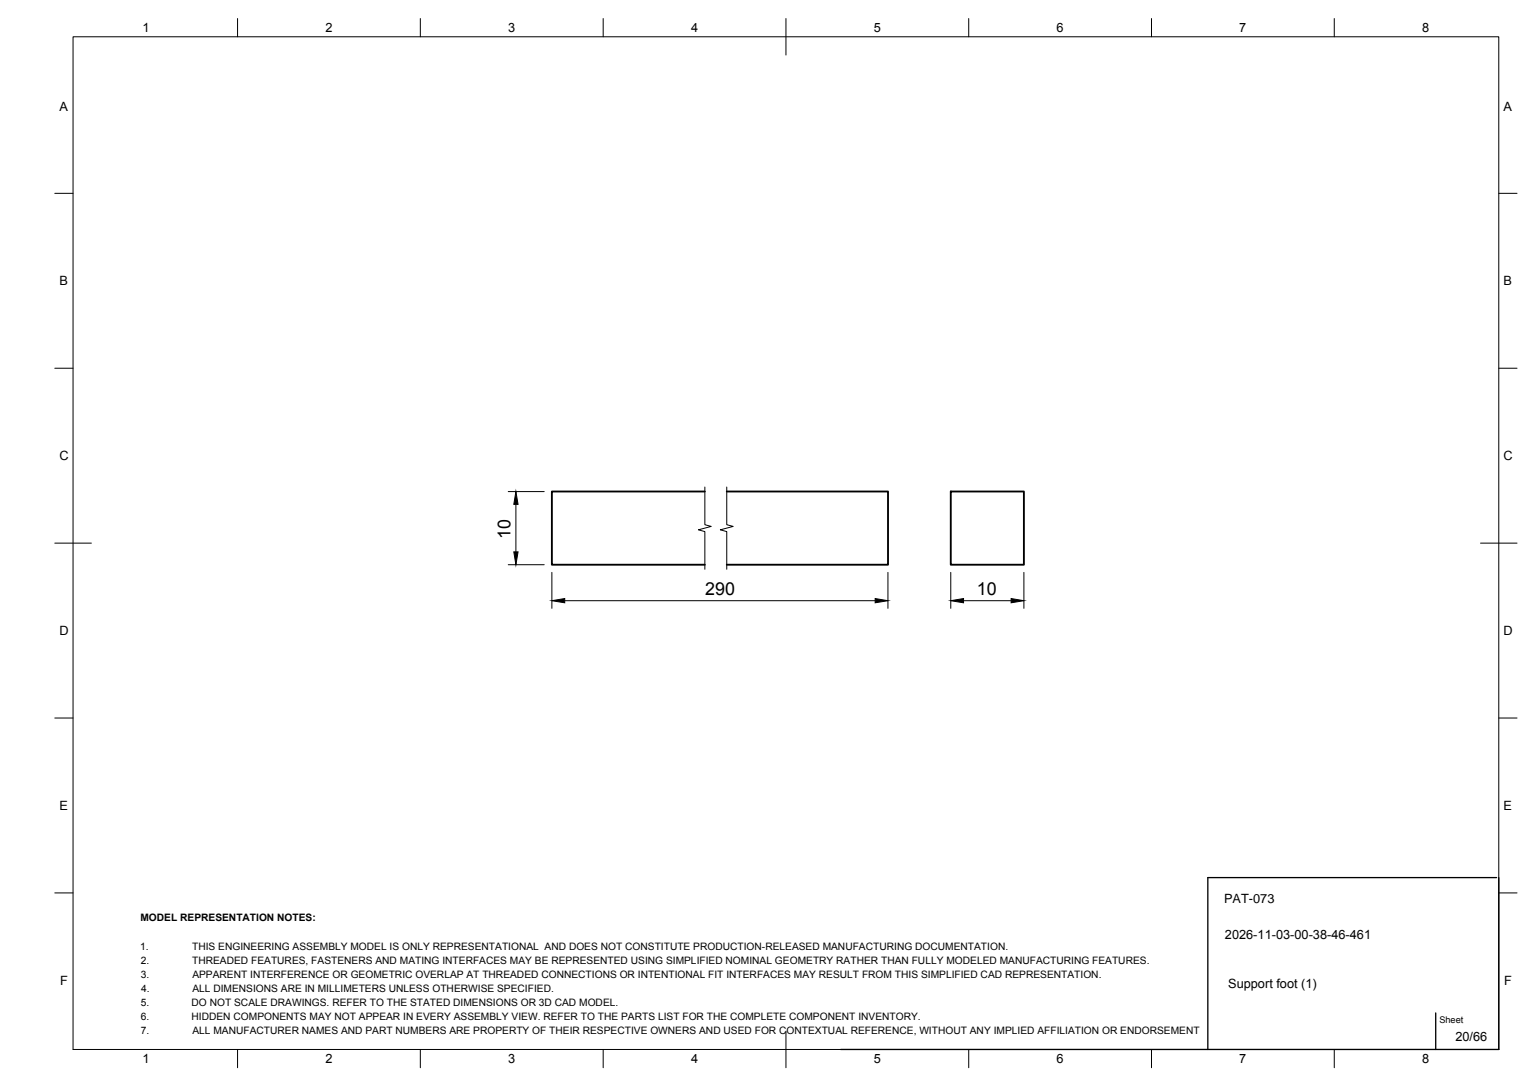
ISO-10303-21;
HEADER;
/* Generated by software containing ST-Developer
 * from STEP Tools, Inc. (www.steptools.com) 
 */

FILE_DESCRIPTION(
/* description */ ('Manual piston pump'),
/* implementation_level */ '2;1');

FILE_NAME(
/* name */ 'Support foot (1).step',
/* time_stamp */ '2026-11-02T16:54:23-08:00',
/* author */ (''),
/* organization */ (''),
/* preprocessor_version */ 'ST-DEVELOPER v20.2',
/* originating_system */ 'Autodesk Translation Framework v15.17.0.0',
/* authorisation */ '');

FILE_SCHEMA (('AUTOMOTIVE_DESIGN { 1 0 10303 214 3 1 1 }'));
ENDSEC;

DATA;
#10=MECHANICAL_DESIGN_GEOMETRIC_PRESENTATION_REPRESENTATION('',(#706),#19043);
#580=SHAPE_REPRESENTATION_RELATIONSHIP('SRR','None',#19326,#643);
#643=ADVANCED_BREP_SHAPE_REPRESENTATION('',(#777),#18993);
#706=STYLED_ITEM('',(#19662),#777);
#777=MANIFOLD_SOLID_BREP('Body1',#9491);
#1462=FACE_OUTER_BOUND('',#2111,.T.);
#1463=FACE_OUTER_BOUND('',#2112,.T.);
#1464=FACE_OUTER_BOUND('',#2113,.T.);
#1465=FACE_OUTER_BOUND('',#2114,.T.);
#1466=FACE_OUTER_BOUND('',#2115,.T.);
#1467=FACE_OUTER_BOUND('',#2116,.T.);
#2111=EDGE_LOOP('',(#6961,#6962,#6963,#6964));
#2112=EDGE_LOOP('',(#6965,#6966,#6967,#6968));
#2113=EDGE_LOOP('',(#6969,#6970,#6971,#6972));
#2114=EDGE_LOOP('',(#6973,#6974,#6975,#6976));
#2115=EDGE_LOOP('',(#6977,#6978,#6979,#6980));
#2116=EDGE_LOOP('',(#6981,#6982,#6983,#6984));
#3337=LINE('',#15442,#3941);
#3338=LINE('',#15444,#3942);
#3339=LINE('',#15446,#3943);
#3340=LINE('',#15447,#3944);
#3341=LINE('',#15450,#3945);
#3342=LINE('',#15452,#3946);
#3343=LINE('',#15453,#3947);
#3344=LINE('',#15456,#3948);
#3345=LINE('',#15458,#3949);
#3346=LINE('',#15459,#3950);
#3347=LINE('',#15461,#3951);
#3348=LINE('',#15462,#3952);
#3941=VECTOR('',#12347,1.);
#3942=VECTOR('',#12348,1.);
#3943=VECTOR('',#12349,1.);
#3944=VECTOR('',#12350,1.);
#3945=VECTOR('',#12353,1.);
#3946=VECTOR('',#12354,1.);
#3947=VECTOR('',#12355,1.);
#3948=VECTOR('',#12358,1.);
#3949=VECTOR('',#12359,1.);
#3950=VECTOR('',#12360,1.);
#3951=VECTOR('',#12363,1.);
#3952=VECTOR('',#12364,1.);
#4581=VERTEX_POINT('',#15440);
#4582=VERTEX_POINT('',#15441);
#4583=VERTEX_POINT('',#15443);
#4584=VERTEX_POINT('',#15445);
#4585=VERTEX_POINT('',#15449);
#4586=VERTEX_POINT('',#15451);
#4587=VERTEX_POINT('',#15455);
#4588=VERTEX_POINT('',#15457);
#5467=EDGE_CURVE('',#4581,#4582,#3337,.T.);
#5468=EDGE_CURVE('',#4582,#4583,#3338,.T.);
#5469=EDGE_CURVE('',#4584,#4583,#3339,.T.);
#5470=EDGE_CURVE('',#4581,#4584,#3340,.T.);
#5471=EDGE_CURVE('',#4585,#4581,#3341,.T.);
#5472=EDGE_CURVE('',#4586,#4584,#3342,.T.);
#5473=EDGE_CURVE('',#4585,#4586,#3343,.T.);
#5474=EDGE_CURVE('',#4587,#4585,#3344,.T.);
#5475=EDGE_CURVE('',#4588,#4586,#3345,.T.);
#5476=EDGE_CURVE('',#4587,#4588,#3346,.T.);
#5477=EDGE_CURVE('',#4582,#4587,#3347,.T.);
#5478=EDGE_CURVE('',#4583,#4588,#3348,.T.);
#6961=ORIENTED_EDGE('',*,*,#5467,.T.);
#6962=ORIENTED_EDGE('',*,*,#5468,.T.);
#6963=ORIENTED_EDGE('',*,*,#5469,.F.);
#6964=ORIENTED_EDGE('',*,*,#5470,.F.);
#6965=ORIENTED_EDGE('',*,*,#5471,.T.);
#6966=ORIENTED_EDGE('',*,*,#5470,.T.);
#6967=ORIENTED_EDGE('',*,*,#5472,.F.);
#6968=ORIENTED_EDGE('',*,*,#5473,.F.);
#6969=ORIENTED_EDGE('',*,*,#5474,.T.);
#6970=ORIENTED_EDGE('',*,*,#5473,.T.);
#6971=ORIENTED_EDGE('',*,*,#5475,.F.);
#6972=ORIENTED_EDGE('',*,*,#5476,.F.);
#6973=ORIENTED_EDGE('',*,*,#5477,.T.);
#6974=ORIENTED_EDGE('',*,*,#5476,.T.);
#6975=ORIENTED_EDGE('',*,*,#5478,.F.);
#6976=ORIENTED_EDGE('',*,*,#5468,.F.);
#6977=ORIENTED_EDGE('',*,*,#5478,.T.);
#6978=ORIENTED_EDGE('',*,*,#5475,.T.);
#6979=ORIENTED_EDGE('',*,*,#5472,.T.);
#6980=ORIENTED_EDGE('',*,*,#5469,.T.);
#6981=ORIENTED_EDGE('',*,*,#5477,.F.);
#6982=ORIENTED_EDGE('',*,*,#5467,.F.);
#6983=ORIENTED_EDGE('',*,*,#5471,.F.);
#6984=ORIENTED_EDGE('',*,*,#5474,.F.);
#8671=PLANE('',#10573);
#8672=PLANE('',#10574);
#8673=PLANE('',#10575);
#8674=PLANE('',#10576);
#8675=PLANE('',#10577);
#8676=PLANE('',#10578);
#9067=ADVANCED_FACE('',(#1462),#8671,.T.);
#9068=ADVANCED_FACE('',(#1463),#8672,.T.);
#9069=ADVANCED_FACE('',(#1464),#8673,.T.);
#9070=ADVANCED_FACE('',(#1465),#8674,.T.);
#9071=ADVANCED_FACE('',(#1466),#8675,.T.);
#9072=ADVANCED_FACE('',(#1467),#8676,.F.);
#9491=CLOSED_SHELL('',(#9067,#9068,#9069,#9070,#9071,#9072));
#10572=AXIS2_PLACEMENT_3D('',#15438,#12343,#12344);
#10573=AXIS2_PLACEMENT_3D('',#15439,#12345,#12346);
#10574=AXIS2_PLACEMENT_3D('',#15448,#12351,#12352);
#10575=AXIS2_PLACEMENT_3D('',#15454,#12356,#12357);
#10576=AXIS2_PLACEMENT_3D('',#15460,#12361,#12362);
#10577=AXIS2_PLACEMENT_3D('',#15463,#12365,#12366);
#10578=AXIS2_PLACEMENT_3D('',#15464,#12367,#12368);
#12343=DIRECTION('axis',(0.,0.,1.));
#12344=DIRECTION('refdir',(1.,0.,0.));
#12345=DIRECTION('center_axis',(0.,1.,0.));
#12346=DIRECTION('ref_axis',(-1.,0.,0.));
#12347=DIRECTION('',(-1.,0.,0.));
#12348=DIRECTION('',(0.,0.,1.));
#12349=DIRECTION('',(-1.,0.,0.));
#12350=DIRECTION('',(0.,0.,1.));
#12351=DIRECTION('center_axis',(1.,0.,0.));
#12352=DIRECTION('ref_axis',(0.,1.,0.));
#12353=DIRECTION('',(0.,1.,0.));
#12354=DIRECTION('',(0.,1.,0.));
#12355=DIRECTION('',(0.,0.,1.));
#12356=DIRECTION('center_axis',(0.,-1.,0.));
#12357=DIRECTION('ref_axis',(1.,0.,0.));
#12358=DIRECTION('',(1.,0.,0.));
#12359=DIRECTION('',(1.,0.,0.));
#12360=DIRECTION('',(0.,0.,1.));
#12361=DIRECTION('center_axis',(-1.,0.,0.));
#12362=DIRECTION('ref_axis',(0.,-1.,0.));
#12363=DIRECTION('',(0.,-1.,0.));
#12364=DIRECTION('',(0.,-1.,0.));
#12365=DIRECTION('center_axis',(0.,0.,1.));
#12366=DIRECTION('ref_axis',(1.,0.,0.));
#12367=DIRECTION('center_axis',(0.,0.,1.));
#12368=DIRECTION('ref_axis',(1.,0.,0.));
#15438=CARTESIAN_POINT('',(0.,0.,0.));
#15439=CARTESIAN_POINT('Origin',(8.5,15.,-2.));
#15440=CARTESIAN_POINT('',(8.5,15.,-2.));
#15441=CARTESIAN_POINT('',(7.5,15.,-2.));
#15442=CARTESIAN_POINT('',(8.5,15.,-2.));
#15443=CARTESIAN_POINT('',(7.5,15.,-1.));
#15444=CARTESIAN_POINT('',(7.5,15.,-2.));
#15445=CARTESIAN_POINT('',(8.5,15.,-1.));
#15446=CARTESIAN_POINT('',(8.5,15.,-1.));
#15447=CARTESIAN_POINT('',(8.5,15.,-2.));
#15448=CARTESIAN_POINT('Origin',(8.5,-14.,-2.));
#15449=CARTESIAN_POINT('',(8.5,-14.,-2.));
#15450=CARTESIAN_POINT('',(8.5,-14.,-2.));
#15451=CARTESIAN_POINT('',(8.5,-14.,-1.));
#15452=CARTESIAN_POINT('',(8.5,-14.,-1.));
#15453=CARTESIAN_POINT('',(8.5,-14.,-2.));
#15454=CARTESIAN_POINT('Origin',(7.5,-14.,-2.));
#15455=CARTESIAN_POINT('',(7.5,-14.,-2.));
#15456=CARTESIAN_POINT('',(7.5,-14.,-2.));
#15457=CARTESIAN_POINT('',(7.5,-14.,-1.));
#15458=CARTESIAN_POINT('',(7.5,-14.,-1.));
#15459=CARTESIAN_POINT('',(7.5,-14.,-2.));
#15460=CARTESIAN_POINT('Origin',(7.5,15.,-2.));
#15461=CARTESIAN_POINT('',(7.5,15.,-2.));
#15462=CARTESIAN_POINT('',(7.5,15.,-1.));
#15463=CARTESIAN_POINT('Origin',(8.,0.5,-1.));
#15464=CARTESIAN_POINT('Origin',(8.,0.5,-2.));
#18922=UNCERTAINTY_MEASURE_WITH_UNIT(LENGTH_MEASURE(0.001),#19044,
'DISTANCE_ACCURACY_VALUE',
'Maximum model space distance between geometric entities at asserted c
onnectivities');
#18972=UNCERTAINTY_MEASURE_WITH_UNIT(LENGTH_MEASURE(0.001),#19044,
'DISTANCE_ACCURACY_VALUE',
'Maximum model space distance between geometric entities at asserted c
onnectivities');
#18993=(
GEOMETRIC_REPRESENTATION_CONTEXT(3)
GLOBAL_UNCERTAINTY_ASSIGNED_CONTEXT((#18922))
GLOBAL_UNIT_ASSIGNED_CONTEXT((#19044,#19046,#19047))
REPRESENTATION_CONTEXT('','3D')
);
#19043=(
GEOMETRIC_REPRESENTATION_CONTEXT(3)
GLOBAL_UNCERTAINTY_ASSIGNED_CONTEXT((#18972))
GLOBAL_UNIT_ASSIGNED_CONTEXT((#19044,#19046,#19047))
REPRESENTATION_CONTEXT('','3D')
);
#19044=(
LENGTH_UNIT()
NAMED_UNIT(*)
SI_UNIT(.CENTI.,.METRE.)
);
#19046=(
NAMED_UNIT(*)
PLANE_ANGLE_UNIT()
SI_UNIT($,.RADIAN.)
);
#19047=(
NAMED_UNIT(*)
SI_UNIT($,.STERADIAN.)
SOLID_ANGLE_UNIT()
);
#19068=SHAPE_DEFINITION_REPRESENTATION(#19138,#19326);
#19138=PRODUCT_DEFINITION_SHAPE('',$,#19397);
#19326=SHAPE_REPRESENTATION('',(#10572),#18993);
#19376=PRODUCT_DEFINITION_CONTEXT('part definition',#19588,'design');
#19397=PRODUCT_DEFINITION('2026-11-03-00-38-46-461','Support foot (1)',
#19467,#19376);
#19467=PRODUCT_DEFINITION_FORMATION('',$,#19610);
#19588=APPLICATION_CONTEXT(
'Core Data for Automotive Mechanical Design Process');
#19589=PRODUCT_CONTEXT('part definition',#19588,'mechanical');
#19610=PRODUCT('2026-11-03-00-38-46-461','Support foot (1)',
'Support foot',(#19589));
#19662=PRESENTATION_STYLE_ASSIGNMENT((#19668));
#19668=SURFACE_STYLE_USAGE(.BOTH.,#19674);
#19674=SURFACE_SIDE_STYLE('',(#19680));
#19680=SURFACE_STYLE_FILL_AREA(#19686);
#19686=FILL_AREA_STYLE('CAD Library Painted - Deep blue',(#19692));
#19692=FILL_AREA_STYLE_COLOUR('CAD Library Painted - Deep blue',#19698);
#19698=COLOUR_RGB('CAD Library Painted - Deep blue',0.0784313725490196,
0.203921568627451,0.349019607843137);
ENDSEC;
END-ISO-10303-21;
